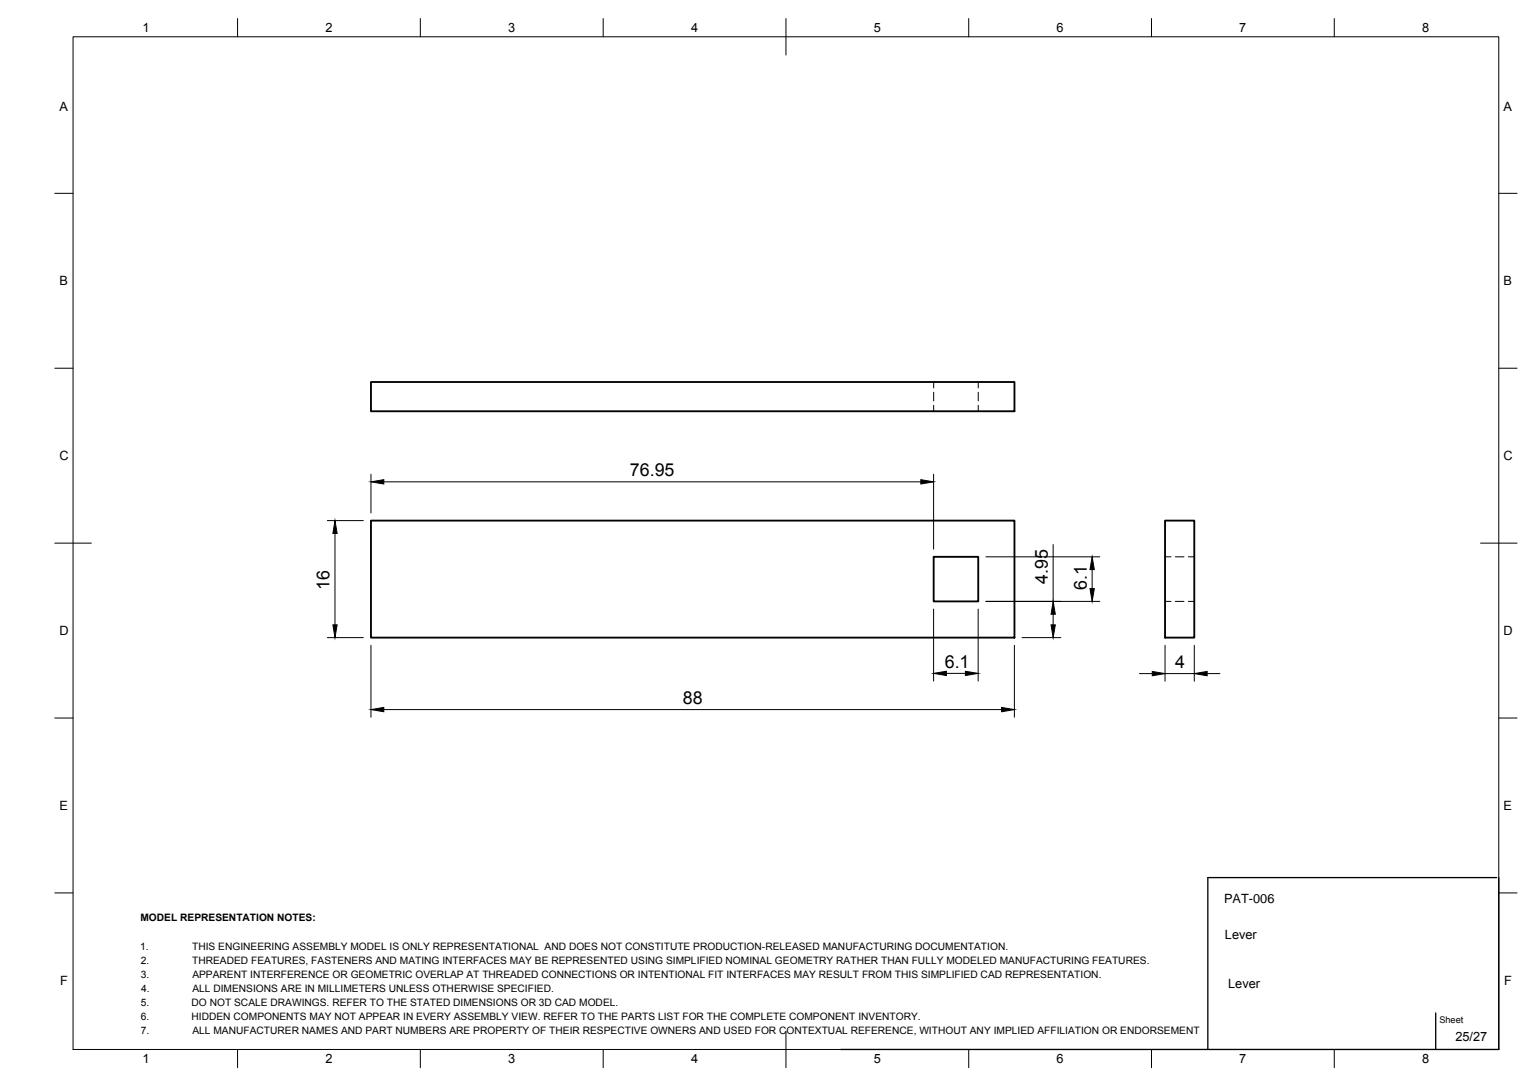
ISO-10303-21;
HEADER;
/* Generated by software containing ST-Developer
 * from STEP Tools, Inc. (www.steptools.com) 
 */

FILE_DESCRIPTION(
/* description */ ('Ball-type isolation valve (generic)'),
/* implementation_level */ '2;1');

FILE_NAME(
/* name */ 'Lever.step',
/* time_stamp */ '2026-10-27T10:53:05-07:00',
/* author */ (''),
/* organization */ (''),
/* preprocessor_version */ 'ST-DEVELOPER v20.2',
/* originating_system */ 'Autodesk Translation Framework v15.17.0.0',
/* authorisation */ '');

FILE_SCHEMA (('AUTOMOTIVE_DESIGN { 1 0 10303 214 3 1 1 }'));
ENDSEC;

DATA;
#10=MECHANICAL_DESIGN_GEOMETRIC_PRESENTATION_REPRESENTATION('',(#299),#7425);
#247=SHAPE_REPRESENTATION_RELATIONSHIP('SRR','None',#7558,#273);
#273=ADVANCED_BREP_SHAPE_REPRESENTATION('',(#323),#7421);
#299=STYLED_ITEM('',(#7758),#323);
#323=MANIFOLD_SOLID_BREP('Body1',#4106);
#414=FACE_BOUND('',#1133,.T.);
#415=FACE_BOUND('',#1135,.T.);
#550=PLANE('',#4838);
#551=PLANE('',#4839);
#552=PLANE('',#4840);
#553=PLANE('',#4841);
#554=PLANE('',#4842);
#555=PLANE('',#4843);
#556=PLANE('',#4844);
#557=PLANE('',#4845);
#558=PLANE('',#4846);
#559=PLANE('',#4847);
#792=FACE_OUTER_BOUND('',#1124,.T.);
#793=FACE_OUTER_BOUND('',#1125,.T.);
#794=FACE_OUTER_BOUND('',#1126,.T.);
#795=FACE_OUTER_BOUND('',#1127,.T.);
#796=FACE_OUTER_BOUND('',#1128,.T.);
#797=FACE_OUTER_BOUND('',#1129,.T.);
#798=FACE_OUTER_BOUND('',#1130,.T.);
#799=FACE_OUTER_BOUND('',#1131,.T.);
#800=FACE_OUTER_BOUND('',#1132,.T.);
#801=FACE_OUTER_BOUND('',#1134,.T.);
#1124=EDGE_LOOP('',(#3621,#3622,#3623,#3624));
#1125=EDGE_LOOP('',(#3625,#3626,#3627,#3628));
#1126=EDGE_LOOP('',(#3629,#3630,#3631,#3632));
#1127=EDGE_LOOP('',(#3633,#3634,#3635,#3636));
#1128=EDGE_LOOP('',(#3637,#3638,#3639,#3640));
#1129=EDGE_LOOP('',(#3641,#3642,#3643,#3644));
#1130=EDGE_LOOP('',(#3645,#3646,#3647,#3648));
#1131=EDGE_LOOP('',(#3649,#3650,#3651,#3652));
#1132=EDGE_LOOP('',(#3653,#3654,#3655,#3656));
#1133=EDGE_LOOP('',(#3657,#3658,#3659,#3660));
#1134=EDGE_LOOP('',(#3661,#3662,#3663,#3664));
#1135=EDGE_LOOP('',(#3665,#3666,#3667,#3668));
#1412=LINE('',#7203,#1720);
#1413=LINE('',#7205,#1721);
#1414=LINE('',#7207,#1722);
#1415=LINE('',#7208,#1723);
#1416=LINE('',#7211,#1724);
#1417=LINE('',#7213,#1725);
#1418=LINE('',#7214,#1726);
#1419=LINE('',#7217,#1727);
#1420=LINE('',#7219,#1728);
#1421=LINE('',#7220,#1729);
#1422=LINE('',#7222,#1730);
#1423=LINE('',#7223,#1731);
#1424=LINE('',#7227,#1732);
#1425=LINE('',#7229,#1733);
#1426=LINE('',#7231,#1734);
#1427=LINE('',#7232,#1735);
#1428=LINE('',#7235,#1736);
#1429=LINE('',#7237,#1737);
#1430=LINE('',#7238,#1738);
#1431=LINE('',#7241,#1739);
#1432=LINE('',#7243,#1740);
#1433=LINE('',#7244,#1741);
#1434=LINE('',#7246,#1742);
#1435=LINE('',#7247,#1743);
#1720=VECTOR('',#6025,1.);
#1721=VECTOR('',#6026,1.);
#1722=VECTOR('',#6027,1.);
#1723=VECTOR('',#6028,1.);
#1724=VECTOR('',#6031,1.);
#1725=VECTOR('',#6032,1.);
#1726=VECTOR('',#6033,1.);
#1727=VECTOR('',#6036,1.);
#1728=VECTOR('',#6037,1.);
#1729=VECTOR('',#6038,1.);
#1730=VECTOR('',#6041,1.);
#1731=VECTOR('',#6042,1.);
#1732=VECTOR('',#6045,1.);
#1733=VECTOR('',#6046,1.);
#1734=VECTOR('',#6047,1.);
#1735=VECTOR('',#6048,1.);
#1736=VECTOR('',#6051,1.);
#1737=VECTOR('',#6052,1.);
#1738=VECTOR('',#6053,1.);
#1739=VECTOR('',#6056,1.);
#1740=VECTOR('',#6057,1.);
#1741=VECTOR('',#6058,1.);
#1742=VECTOR('',#6061,1.);
#1743=VECTOR('',#6062,1.);
#2233=VERTEX_POINT('',#7201);
#2234=VERTEX_POINT('',#7202);
#2235=VERTEX_POINT('',#7204);
#2236=VERTEX_POINT('',#7206);
#2237=VERTEX_POINT('',#7210);
#2238=VERTEX_POINT('',#7212);
#2239=VERTEX_POINT('',#7216);
#2240=VERTEX_POINT('',#7218);
#2241=VERTEX_POINT('',#7225);
#2242=VERTEX_POINT('',#7226);
#2243=VERTEX_POINT('',#7228);
#2244=VERTEX_POINT('',#7230);
#2245=VERTEX_POINT('',#7234);
#2246=VERTEX_POINT('',#7236);
#2247=VERTEX_POINT('',#7240);
#2248=VERTEX_POINT('',#7242);
#2703=EDGE_CURVE('',#2233,#2234,#1412,.T.);
#2704=EDGE_CURVE('',#2235,#2233,#1413,.T.);
#2705=EDGE_CURVE('',#2236,#2235,#1414,.T.);
#2706=EDGE_CURVE('',#2236,#2234,#1415,.T.);
#2707=EDGE_CURVE('',#2234,#2237,#1416,.T.);
#2708=EDGE_CURVE('',#2238,#2236,#1417,.T.);
#2709=EDGE_CURVE('',#2238,#2237,#1418,.T.);
#2710=EDGE_CURVE('',#2237,#2239,#1419,.T.);
#2711=EDGE_CURVE('',#2240,#2238,#1420,.T.);
#2712=EDGE_CURVE('',#2240,#2239,#1421,.T.);
#2713=EDGE_CURVE('',#2239,#2233,#1422,.T.);
#2714=EDGE_CURVE('',#2235,#2240,#1423,.T.);
#2715=EDGE_CURVE('',#2241,#2242,#1424,.T.);
#2716=EDGE_CURVE('',#2242,#2243,#1425,.T.);
#2717=EDGE_CURVE('',#2244,#2243,#1426,.T.);
#2718=EDGE_CURVE('',#2241,#2244,#1427,.T.);
#2719=EDGE_CURVE('',#2245,#2241,#1428,.T.);
#2720=EDGE_CURVE('',#2246,#2244,#1429,.T.);
#2721=EDGE_CURVE('',#2245,#2246,#1430,.T.);
#2722=EDGE_CURVE('',#2247,#2245,#1431,.T.);
#2723=EDGE_CURVE('',#2248,#2246,#1432,.T.);
#2724=EDGE_CURVE('',#2247,#2248,#1433,.T.);
#2725=EDGE_CURVE('',#2242,#2247,#1434,.T.);
#2726=EDGE_CURVE('',#2243,#2248,#1435,.T.);
#3621=ORIENTED_EDGE('',*,*,#2703,.F.);
#3622=ORIENTED_EDGE('',*,*,#2704,.F.);
#3623=ORIENTED_EDGE('',*,*,#2705,.F.);
#3624=ORIENTED_EDGE('',*,*,#2706,.T.);
#3625=ORIENTED_EDGE('',*,*,#2707,.F.);
#3626=ORIENTED_EDGE('',*,*,#2706,.F.);
#3627=ORIENTED_EDGE('',*,*,#2708,.F.);
#3628=ORIENTED_EDGE('',*,*,#2709,.T.);
#3629=ORIENTED_EDGE('',*,*,#2710,.F.);
#3630=ORIENTED_EDGE('',*,*,#2709,.F.);
#3631=ORIENTED_EDGE('',*,*,#2711,.F.);
#3632=ORIENTED_EDGE('',*,*,#2712,.T.);
#3633=ORIENTED_EDGE('',*,*,#2713,.F.);
#3634=ORIENTED_EDGE('',*,*,#2712,.F.);
#3635=ORIENTED_EDGE('',*,*,#2714,.F.);
#3636=ORIENTED_EDGE('',*,*,#2704,.T.);
#3637=ORIENTED_EDGE('',*,*,#2715,.T.);
#3638=ORIENTED_EDGE('',*,*,#2716,.T.);
#3639=ORIENTED_EDGE('',*,*,#2717,.F.);
#3640=ORIENTED_EDGE('',*,*,#2718,.F.);
#3641=ORIENTED_EDGE('',*,*,#2719,.T.);
#3642=ORIENTED_EDGE('',*,*,#2718,.T.);
#3643=ORIENTED_EDGE('',*,*,#2720,.F.);
#3644=ORIENTED_EDGE('',*,*,#2721,.F.);
#3645=ORIENTED_EDGE('',*,*,#2722,.T.);
#3646=ORIENTED_EDGE('',*,*,#2721,.T.);
#3647=ORIENTED_EDGE('',*,*,#2723,.F.);
#3648=ORIENTED_EDGE('',*,*,#2724,.F.);
#3649=ORIENTED_EDGE('',*,*,#2725,.T.);
#3650=ORIENTED_EDGE('',*,*,#2724,.T.);
#3651=ORIENTED_EDGE('',*,*,#2726,.F.);
#3652=ORIENTED_EDGE('',*,*,#2716,.F.);
#3653=ORIENTED_EDGE('',*,*,#2726,.T.);
#3654=ORIENTED_EDGE('',*,*,#2723,.T.);
#3655=ORIENTED_EDGE('',*,*,#2720,.T.);
#3656=ORIENTED_EDGE('',*,*,#2717,.T.);
#3657=ORIENTED_EDGE('',*,*,#2710,.T.);
#3658=ORIENTED_EDGE('',*,*,#2713,.T.);
#3659=ORIENTED_EDGE('',*,*,#2703,.T.);
#3660=ORIENTED_EDGE('',*,*,#2707,.T.);
#3661=ORIENTED_EDGE('',*,*,#2725,.F.);
#3662=ORIENTED_EDGE('',*,*,#2715,.F.);
#3663=ORIENTED_EDGE('',*,*,#2719,.F.);
#3664=ORIENTED_EDGE('',*,*,#2722,.F.);
#3665=ORIENTED_EDGE('',*,*,#2711,.T.);
#3666=ORIENTED_EDGE('',*,*,#2708,.T.);
#3667=ORIENTED_EDGE('',*,*,#2705,.T.);
#3668=ORIENTED_EDGE('',*,*,#2714,.T.);
#4046=ADVANCED_FACE('',(#792),#550,.F.);
#4047=ADVANCED_FACE('',(#793),#551,.F.);
#4048=ADVANCED_FACE('',(#794),#552,.F.);
#4049=ADVANCED_FACE('',(#795),#553,.F.);
#4050=ADVANCED_FACE('',(#796),#554,.T.);
#4051=ADVANCED_FACE('',(#797),#555,.T.);
#4052=ADVANCED_FACE('',(#798),#556,.T.);
#4053=ADVANCED_FACE('',(#799),#557,.T.);
#4054=ADVANCED_FACE('',(#800,#414),#558,.T.);
#4055=ADVANCED_FACE('',(#801,#415),#559,.F.);
#4106=CLOSED_SHELL('',(#4046,#4047,#4048,#4049,#4050,#4051,#4052,#4053,
#4054,#4055));
#4837=AXIS2_PLACEMENT_3D('',#7199,#6021,#6022);
#4838=AXIS2_PLACEMENT_3D('',#7200,#6023,#6024);
#4839=AXIS2_PLACEMENT_3D('',#7209,#6029,#6030);
#4840=AXIS2_PLACEMENT_3D('',#7215,#6034,#6035);
#4841=AXIS2_PLACEMENT_3D('',#7221,#6039,#6040);
#4842=AXIS2_PLACEMENT_3D('',#7224,#6043,#6044);
#4843=AXIS2_PLACEMENT_3D('',#7233,#6049,#6050);
#4844=AXIS2_PLACEMENT_3D('',#7239,#6054,#6055);
#4845=AXIS2_PLACEMENT_3D('',#7245,#6059,#6060);
#4846=AXIS2_PLACEMENT_3D('',#7248,#6063,#6064);
#4847=AXIS2_PLACEMENT_3D('',#7249,#6065,#6066);
#6021=DIRECTION('axis',(0.,0.,1.));
#6022=DIRECTION('refdir',(1.,0.,0.));
#6023=DIRECTION('center_axis',(0.,-1.,0.));
#6024=DIRECTION('ref_axis',(1.,0.,0.));
#6025=DIRECTION('',(-1.,0.,0.));
#6026=DIRECTION('',(0.,0.,1.));
#6027=DIRECTION('',(1.,0.,0.));
#6028=DIRECTION('',(0.,0.,1.));
#6029=DIRECTION('center_axis',(-1.,0.,0.));
#6030=DIRECTION('ref_axis',(0.,-1.,0.));
#6031=DIRECTION('',(0.,1.,0.));
#6032=DIRECTION('',(0.,-1.,0.));
#6033=DIRECTION('',(0.,0.,1.));
#6034=DIRECTION('center_axis',(0.,1.,0.));
#6035=DIRECTION('ref_axis',(-1.,0.,0.));
#6036=DIRECTION('',(1.,0.,0.));
#6037=DIRECTION('',(-1.,0.,0.));
#6038=DIRECTION('',(0.,0.,1.));
#6039=DIRECTION('center_axis',(1.,0.,0.));
#6040=DIRECTION('ref_axis',(0.,1.,0.));
#6041=DIRECTION('',(0.,-1.,0.));
#6042=DIRECTION('',(0.,1.,0.));
#6043=DIRECTION('center_axis',(0.,1.,0.));
#6044=DIRECTION('ref_axis',(-1.,0.,0.));
#6045=DIRECTION('',(-1.,0.,0.));
#6046=DIRECTION('',(0.,0.,1.));
#6047=DIRECTION('',(-1.,0.,0.));
#6048=DIRECTION('',(0.,0.,1.));
#6049=DIRECTION('center_axis',(1.,0.,0.));
#6050=DIRECTION('ref_axis',(0.,1.,0.));
#6051=DIRECTION('',(0.,1.,0.));
#6052=DIRECTION('',(0.,1.,0.));
#6053=DIRECTION('',(0.,0.,1.));
#6054=DIRECTION('center_axis',(0.,-1.,0.));
#6055=DIRECTION('ref_axis',(1.,0.,0.));
#6056=DIRECTION('',(1.,0.,0.));
#6057=DIRECTION('',(1.,0.,0.));
#6058=DIRECTION('',(0.,0.,1.));
#6059=DIRECTION('center_axis',(-1.,0.,0.));
#6060=DIRECTION('ref_axis',(0.,-1.,0.));
#6061=DIRECTION('',(0.,-1.,0.));
#6062=DIRECTION('',(0.,-1.,0.));
#6063=DIRECTION('center_axis',(0.,0.,1.));
#6064=DIRECTION('ref_axis',(1.,0.,0.));
#6065=DIRECTION('center_axis',(0.,0.,1.));
#6066=DIRECTION('ref_axis',(1.,0.,0.));
#7199=CARTESIAN_POINT('',(0.,0.,0.));
#7200=CARTESIAN_POINT('Origin',(-0.305,-0.305,8.9));
#7201=CARTESIAN_POINT('',(0.305,-0.305,9.4));
#7202=CARTESIAN_POINT('',(-0.305,-0.305,9.4));
#7203=CARTESIAN_POINT('',(1.6475,-0.305,9.4));
#7204=CARTESIAN_POINT('',(0.305,-0.305,9.));
#7205=CARTESIAN_POINT('',(0.305,-0.305,8.9));
#7206=CARTESIAN_POINT('',(-0.305,-0.305,9.));
#7207=CARTESIAN_POINT('',(1.6475,-0.305,9.));
#7208=CARTESIAN_POINT('',(-0.305,-0.305,8.9));
#7209=CARTESIAN_POINT('Origin',(-0.305,0.305,8.9));
#7210=CARTESIAN_POINT('',(-0.305,0.305,9.4));
#7211=CARTESIAN_POINT('',(-0.305,0.1525,9.4));
#7212=CARTESIAN_POINT('',(-0.305,0.305,9.));
#7213=CARTESIAN_POINT('',(-0.305,0.1525,9.));
#7214=CARTESIAN_POINT('',(-0.305,0.305,8.9));
#7215=CARTESIAN_POINT('Origin',(0.305,0.305,8.9));
#7216=CARTESIAN_POINT('',(0.305,0.305,9.4));
#7217=CARTESIAN_POINT('',(1.9525,0.305,9.4));
#7218=CARTESIAN_POINT('',(0.305,0.305,9.));
#7219=CARTESIAN_POINT('',(1.9525,0.305,9.));
#7220=CARTESIAN_POINT('',(0.305,0.305,8.9));
#7221=CARTESIAN_POINT('Origin',(0.305,-0.305,8.9));
#7222=CARTESIAN_POINT('',(0.305,-0.1525,9.4));
#7223=CARTESIAN_POINT('',(0.305,-0.1525,9.));
#7224=CARTESIAN_POINT('Origin',(8.,0.8,9.));
#7225=CARTESIAN_POINT('',(8.,0.8,9.));
#7226=CARTESIAN_POINT('',(-0.8,0.8,9.));
#7227=CARTESIAN_POINT('',(8.,0.8,9.));
#7228=CARTESIAN_POINT('',(-0.8,0.8,9.4));
#7229=CARTESIAN_POINT('',(-0.8,0.8,9.));
#7230=CARTESIAN_POINT('',(8.,0.8,9.4));
#7231=CARTESIAN_POINT('',(8.,0.8,9.4));
#7232=CARTESIAN_POINT('',(8.,0.8,9.));
#7233=CARTESIAN_POINT('Origin',(8.,-0.8,9.));
#7234=CARTESIAN_POINT('',(8.,-0.8,9.));
#7235=CARTESIAN_POINT('',(8.,-0.8,9.));
#7236=CARTESIAN_POINT('',(8.,-0.8,9.4));
#7237=CARTESIAN_POINT('',(8.,-0.8,9.4));
#7238=CARTESIAN_POINT('',(8.,-0.8,9.));
#7239=CARTESIAN_POINT('Origin',(-0.8,-0.8,9.));
#7240=CARTESIAN_POINT('',(-0.8,-0.8,9.));
#7241=CARTESIAN_POINT('',(-0.8,-0.8,9.));
#7242=CARTESIAN_POINT('',(-0.8,-0.8,9.4));
#7243=CARTESIAN_POINT('',(-0.8,-0.8,9.4));
#7244=CARTESIAN_POINT('',(-0.8,-0.8,9.));
#7245=CARTESIAN_POINT('Origin',(-0.8,0.8,9.));
#7246=CARTESIAN_POINT('',(-0.8,0.8,9.));
#7247=CARTESIAN_POINT('',(-0.8,0.8,9.4));
#7248=CARTESIAN_POINT('Origin',(3.6,0.,9.4));
#7249=CARTESIAN_POINT('Origin',(3.6,0.,9.));
#7391=UNCERTAINTY_MEASURE_WITH_UNIT(LENGTH_MEASURE(0.001),#7426,
'DISTANCE_ACCURACY_VALUE',
'Maximum model space distance between geometric entities at asserted c
onnectivities');
#7395=UNCERTAINTY_MEASURE_WITH_UNIT(LENGTH_MEASURE(0.001),#7426,
'DISTANCE_ACCURACY_VALUE',
'Maximum model space distance between geometric entities at asserted c
onnectivities');
#7421=(
GEOMETRIC_REPRESENTATION_CONTEXT(3)
GLOBAL_UNCERTAINTY_ASSIGNED_CONTEXT((#7391))
GLOBAL_UNIT_ASSIGNED_CONTEXT((#7426,#7428,#7429))
REPRESENTATION_CONTEXT('','3D')
);
#7425=(
GEOMETRIC_REPRESENTATION_CONTEXT(3)
GLOBAL_UNCERTAINTY_ASSIGNED_CONTEXT((#7395))
GLOBAL_UNIT_ASSIGNED_CONTEXT((#7426,#7428,#7429))
REPRESENTATION_CONTEXT('','3D')
);
#7426=(
LENGTH_UNIT()
NAMED_UNIT(*)
SI_UNIT(.CENTI.,.METRE.)
);
#7428=(
NAMED_UNIT(*)
PLANE_ANGLE_UNIT()
SI_UNIT($,.RADIAN.)
);
#7429=(
NAMED_UNIT(*)
SI_UNIT($,.STERADIAN.)
SOLID_ANGLE_UNIT()
);
#7455=SHAPE_DEFINITION_REPRESENTATION(#7521,#7558);
#7521=PRODUCT_DEFINITION_SHAPE('',$,#7588);
#7558=SHAPE_REPRESENTATION('',(#4837),#7421);
#7562=PRODUCT_DEFINITION_CONTEXT('part definition',#7651,'design');
#7588=PRODUCT_DEFINITION('Lever','Lever',#7617,#7562);
#7617=PRODUCT_DEFINITION_FORMATION('',$,#7678);
#7651=APPLICATION_CONTEXT(
'Core Data for Automotive Mechanical Design Process');
#7652=PRODUCT_CONTEXT('part definition',#7651,'mechanical');
#7678=PRODUCT('Lever','Lever','Lever',(#7652));
#7752=COLOUR_RGB('Off White',0.89,0.88,0.83);
#7753=FILL_AREA_STYLE_COLOUR('',#7752);
#7754=FILL_AREA_STYLE('',(#7753));
#7755=SURFACE_STYLE_FILL_AREA(#7754);
#7756=SURFACE_SIDE_STYLE('',(#7755));
#7757=SURFACE_STYLE_USAGE(.BOTH.,#7756);
#7758=PRESENTATION_STYLE_ASSIGNMENT((#7757));
ENDSEC;
END-ISO-10303-21;
